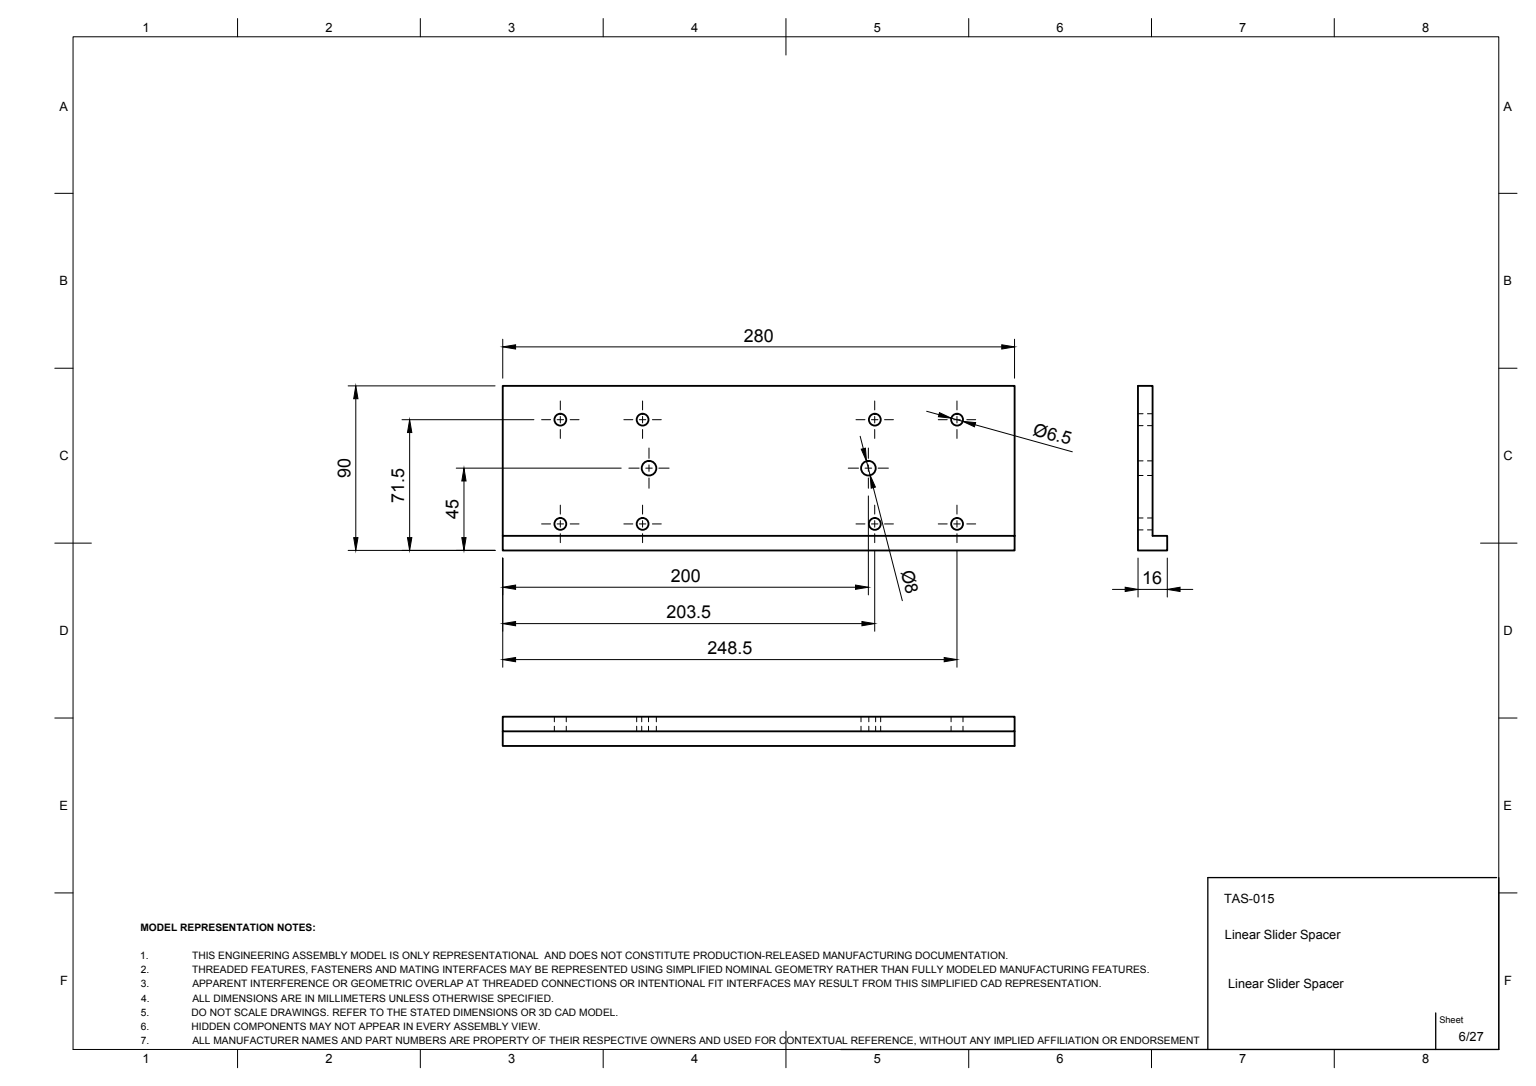
ISO-10303-21;
HEADER;
/* Generated by software containing ST-Developer
 * from STEP Tools, Inc. (www.steptools.com) 
 */

FILE_DESCRIPTION(
/* description */ ('STEP AP214'),
/* implementation_level */ '2;1');

FILE_NAME(
/* name */ 'Linear Slider Spacer.step',
/* time_stamp */ '2026-11-15T14:49:54-08:00',
/* author */ (''),
/* organization */ (''),
/* preprocessor_version */ 'ST-DEVELOPER v20.2',
/* originating_system */ 'Autodesk Translation Framework v15.17.0.0',
/* authorisation */ '');

FILE_SCHEMA (('AUTOMOTIVE_DESIGN { 1 0 10303 214 3 1 1 }'));
ENDSEC;

DATA;
#10=MECHANICAL_DESIGN_GEOMETRIC_PRESENTATION_REPRESENTATION('',(#1131),#66721);
#1065=SHAPE_REPRESENTATION_RELATIONSHIP('SRR','None',#66928,#1096);
#1096=ADVANCED_BREP_SHAPE_REPRESENTATION('',(#1166),#66719);
#1131=STYLED_ITEM('',(#67095),#1166);
#1166=MANIFOLD_SOLID_BREP('Body1',#25697);
#1476=FACE_BOUND('',#5440,.T.);
#1477=FACE_BOUND('',#5441,.T.);
#1478=FACE_BOUND('',#5442,.T.);
#1479=FACE_BOUND('',#5443,.T.);
#1480=FACE_BOUND('',#5444,.T.);
#1481=FACE_BOUND('',#5445,.T.);
#1482=FACE_BOUND('',#5446,.T.);
#1483=FACE_BOUND('',#5447,.T.);
#1484=FACE_BOUND('',#5448,.T.);
#1485=FACE_BOUND('',#5449,.T.);
#1486=FACE_BOUND('',#5455,.T.);
#1487=FACE_BOUND('',#5456,.T.);
#1488=FACE_BOUND('',#5457,.T.);
#1489=FACE_BOUND('',#5458,.T.);
#1490=FACE_BOUND('',#5459,.T.);
#1491=FACE_BOUND('',#5460,.T.);
#1492=FACE_BOUND('',#5461,.T.);
#1493=FACE_BOUND('',#5462,.T.);
#1494=FACE_BOUND('',#5463,.T.);
#1495=FACE_BOUND('',#5464,.T.);
#2251=PLANE('',#28672);
#2252=PLANE('',#28673);
#2253=PLANE('',#28674);
#2254=PLANE('',#28675);
#2255=PLANE('',#28676);
#2256=PLANE('',#28677);
#2257=PLANE('',#28678);
#2258=PLANE('',#28679);
#3679=FACE_OUTER_BOUND('',#5429,.T.);
#3680=FACE_OUTER_BOUND('',#5430,.T.);
#3681=FACE_OUTER_BOUND('',#5431,.T.);
#3682=FACE_OUTER_BOUND('',#5432,.T.);
#3683=FACE_OUTER_BOUND('',#5433,.T.);
#3684=FACE_OUTER_BOUND('',#5434,.T.);
#3685=FACE_OUTER_BOUND('',#5435,.T.);
#3686=FACE_OUTER_BOUND('',#5436,.T.);
#3687=FACE_OUTER_BOUND('',#5437,.T.);
#3688=FACE_OUTER_BOUND('',#5438,.T.);
#3689=FACE_OUTER_BOUND('',#5439,.T.);
#3690=FACE_OUTER_BOUND('',#5450,.T.);
#3691=FACE_OUTER_BOUND('',#5451,.T.);
#3692=FACE_OUTER_BOUND('',#5452,.T.);
#3693=FACE_OUTER_BOUND('',#5453,.T.);
#3694=FACE_OUTER_BOUND('',#5454,.T.);
#3695=FACE_OUTER_BOUND('',#5465,.T.);
#3696=FACE_OUTER_BOUND('',#5466,.T.);
#5429=EDGE_LOOP('',(#23648,#23649,#23650,#23651));
#5430=EDGE_LOOP('',(#23652,#23653,#23654,#23655));
#5431=EDGE_LOOP('',(#23656,#23657,#23658,#23659));
#5432=EDGE_LOOP('',(#23660,#23661,#23662,#23663));
#5433=EDGE_LOOP('',(#23664,#23665,#23666,#23667));
#5434=EDGE_LOOP('',(#23668,#23669,#23670,#23671));
#5435=EDGE_LOOP('',(#23672,#23673,#23674,#23675));
#5436=EDGE_LOOP('',(#23676,#23677,#23678,#23679));
#5437=EDGE_LOOP('',(#23680,#23681,#23682,#23683));
#5438=EDGE_LOOP('',(#23684,#23685,#23686,#23687));
#5439=EDGE_LOOP('',(#23688,#23689,#23690,#23691));
#5440=EDGE_LOOP('',(#23692));
#5441=EDGE_LOOP('',(#23693));
#5442=EDGE_LOOP('',(#23694));
#5443=EDGE_LOOP('',(#23695));
#5444=EDGE_LOOP('',(#23696));
#5445=EDGE_LOOP('',(#23697));
#5446=EDGE_LOOP('',(#23698));
#5447=EDGE_LOOP('',(#23699));
#5448=EDGE_LOOP('',(#23700));
#5449=EDGE_LOOP('',(#23701));
#5450=EDGE_LOOP('',(#23702,#23703,#23704,#23705));
#5451=EDGE_LOOP('',(#23706,#23707,#23708,#23709,#23710,#23711));
#5452=EDGE_LOOP('',(#23712,#23713,#23714,#23715));
#5453=EDGE_LOOP('',(#23716,#23717,#23718,#23719,#23720,#23721));
#5454=EDGE_LOOP('',(#23722,#23723,#23724,#23725));
#5455=EDGE_LOOP('',(#23726));
#5456=EDGE_LOOP('',(#23727));
#5457=EDGE_LOOP('',(#23728));
#5458=EDGE_LOOP('',(#23729));
#5459=EDGE_LOOP('',(#23730));
#5460=EDGE_LOOP('',(#23731));
#5461=EDGE_LOOP('',(#23732));
#5462=EDGE_LOOP('',(#23733));
#5463=EDGE_LOOP('',(#23734));
#5464=EDGE_LOOP('',(#23735));
#5465=EDGE_LOOP('',(#23736,#23737,#23738,#23739));
#5466=EDGE_LOOP('',(#23740,#23741,#23742,#23743));
#7422=LINE('',#66429,#9411);
#7423=LINE('',#66435,#9412);
#7424=LINE('',#66441,#9413);
#7425=LINE('',#66447,#9414);
#7426=LINE('',#66453,#9415);
#7427=LINE('',#66459,#9416);
#7428=LINE('',#66465,#9417);
#7429=LINE('',#66471,#9418);
#7430=LINE('',#66477,#9419);
#7431=LINE('',#66483,#9420);
#7432=LINE('',#66488,#9421);
#7433=LINE('',#66490,#9422);
#7434=LINE('',#66492,#9423);
#7435=LINE('',#66493,#9424);
#7436=LINE('',#66496,#9425);
#7437=LINE('',#66498,#9426);
#7438=LINE('',#66499,#9427);
#7439=LINE('',#66502,#9428);
#7440=LINE('',#66504,#9429);
#7441=LINE('',#66506,#9430);
#7442=LINE('',#66507,#9431);
#7443=LINE('',#66510,#9432);
#7444=LINE('',#66512,#9433);
#7445=LINE('',#66513,#9434);
#7446=LINE('',#66516,#9435);
#7447=LINE('',#66517,#9436);
#7448=LINE('',#66518,#9437);
#7449=LINE('',#66521,#9438);
#9411=VECTOR('',#35901,4.);
#9412=VECTOR('',#35908,4.);
#9413=VECTOR('',#35915,3.25);
#9414=VECTOR('',#35922,3.25);
#9415=VECTOR('',#35929,3.25);
#9416=VECTOR('',#35936,3.25);
#9417=VECTOR('',#35943,3.25);
#9418=VECTOR('',#35950,3.25);
#9419=VECTOR('',#35957,3.25);
#9420=VECTOR('',#35964,3.25);
#9421=VECTOR('',#35969,1000.);
#9422=VECTOR('',#35970,1000.);
#9423=VECTOR('',#35971,1000.);
#9424=VECTOR('',#35972,1000.);
#9425=VECTOR('',#35975,1000.);
#9426=VECTOR('',#35976,1000.);
#9427=VECTOR('',#35977,1000.);
#9428=VECTOR('',#35980,1000.);
#9429=VECTOR('',#35981,1000.);
#9430=VECTOR('',#35982,1000.);
#9431=VECTOR('',#35983,1000.);
#9432=VECTOR('',#35986,1000.);
#9433=VECTOR('',#35987,1000.);
#9434=VECTOR('',#35988,1000.);
#9435=VECTOR('',#35991,1000.);
#9436=VECTOR('',#35992,1000.);
#9437=VECTOR('',#35993,1000.);
#9438=VECTOR('',#35998,1000.);
#10611=CIRCLE('',#28643,4.);
#10612=CIRCLE('',#28644,4.);
#10613=CIRCLE('',#28646,4.);
#10614=CIRCLE('',#28647,4.);
#10615=CIRCLE('',#28649,3.25);
#10616=CIRCLE('',#28650,3.25);
#10617=CIRCLE('',#28652,3.25);
#10618=CIRCLE('',#28653,3.25);
#10619=CIRCLE('',#28655,3.25);
#10620=CIRCLE('',#28656,3.25);
#10621=CIRCLE('',#28658,3.25);
#10622=CIRCLE('',#28659,3.25);
#10623=CIRCLE('',#28661,3.25);
#10624=CIRCLE('',#28662,3.25);
#10625=CIRCLE('',#28664,3.25);
#10626=CIRCLE('',#28665,3.25);
#10627=CIRCLE('',#28667,3.25);
#10628=CIRCLE('',#28668,3.25);
#10629=CIRCLE('',#28670,3.25);
#10630=CIRCLE('',#28671,3.25);
#12939=VERTEX_POINT('',#66426);
#12940=VERTEX_POINT('',#66428);
#12941=VERTEX_POINT('',#66432);
#12942=VERTEX_POINT('',#66434);
#12943=VERTEX_POINT('',#66438);
#12944=VERTEX_POINT('',#66440);
#12945=VERTEX_POINT('',#66444);
#12946=VERTEX_POINT('',#66446);
#12947=VERTEX_POINT('',#66450);
#12948=VERTEX_POINT('',#66452);
#12949=VERTEX_POINT('',#66456);
#12950=VERTEX_POINT('',#66458);
#12951=VERTEX_POINT('',#66462);
#12952=VERTEX_POINT('',#66464);
#12953=VERTEX_POINT('',#66468);
#12954=VERTEX_POINT('',#66470);
#12955=VERTEX_POINT('',#66474);
#12956=VERTEX_POINT('',#66476);
#12957=VERTEX_POINT('',#66480);
#12958=VERTEX_POINT('',#66482);
#12959=VERTEX_POINT('',#66486);
#12960=VERTEX_POINT('',#66487);
#12961=VERTEX_POINT('',#66489);
#12962=VERTEX_POINT('',#66491);
#12963=VERTEX_POINT('',#66495);
#12964=VERTEX_POINT('',#66497);
#12965=VERTEX_POINT('',#66501);
#12966=VERTEX_POINT('',#66503);
#12967=VERTEX_POINT('',#66505);
#12968=VERTEX_POINT('',#66509);
#12969=VERTEX_POINT('',#66511);
#12970=VERTEX_POINT('',#66515);
#16517=EDGE_CURVE('',#12939,#12939,#10611,.T.);
#16518=EDGE_CURVE('',#12939,#12940,#7422,.T.);
#16519=EDGE_CURVE('',#12940,#12940,#10612,.T.);
#16520=EDGE_CURVE('',#12941,#12941,#10613,.T.);
#16521=EDGE_CURVE('',#12941,#12942,#7423,.T.);
#16522=EDGE_CURVE('',#12942,#12942,#10614,.T.);
#16523=EDGE_CURVE('',#12943,#12943,#10615,.T.);
#16524=EDGE_CURVE('',#12943,#12944,#7424,.T.);
#16525=EDGE_CURVE('',#12944,#12944,#10616,.T.);
#16526=EDGE_CURVE('',#12945,#12945,#10617,.T.);
#16527=EDGE_CURVE('',#12945,#12946,#7425,.T.);
#16528=EDGE_CURVE('',#12946,#12946,#10618,.T.);
#16529=EDGE_CURVE('',#12947,#12947,#10619,.T.);
#16530=EDGE_CURVE('',#12947,#12948,#7426,.T.);
#16531=EDGE_CURVE('',#12948,#12948,#10620,.T.);
#16532=EDGE_CURVE('',#12949,#12949,#10621,.T.);
#16533=EDGE_CURVE('',#12949,#12950,#7427,.T.);
#16534=EDGE_CURVE('',#12950,#12950,#10622,.T.);
#16535=EDGE_CURVE('',#12951,#12951,#10623,.T.);
#16536=EDGE_CURVE('',#12951,#12952,#7428,.T.);
#16537=EDGE_CURVE('',#12952,#12952,#10624,.T.);
#16538=EDGE_CURVE('',#12953,#12953,#10625,.T.);
#16539=EDGE_CURVE('',#12953,#12954,#7429,.T.);
#16540=EDGE_CURVE('',#12954,#12954,#10626,.T.);
#16541=EDGE_CURVE('',#12955,#12955,#10627,.T.);
#16542=EDGE_CURVE('',#12955,#12956,#7430,.T.);
#16543=EDGE_CURVE('',#12956,#12956,#10628,.T.);
#16544=EDGE_CURVE('',#12957,#12957,#10629,.T.);
#16545=EDGE_CURVE('',#12957,#12958,#7431,.T.);
#16546=EDGE_CURVE('',#12958,#12958,#10630,.T.);
#16547=EDGE_CURVE('',#12959,#12960,#7432,.T.);
#16548=EDGE_CURVE('',#12961,#12959,#7433,.T.);
#16549=EDGE_CURVE('',#12962,#12961,#7434,.T.);
#16550=EDGE_CURVE('',#12960,#12962,#7435,.T.);
#16551=EDGE_CURVE('',#12963,#12961,#7436,.T.);
#16552=EDGE_CURVE('',#12964,#12963,#7437,.T.);
#16553=EDGE_CURVE('',#12964,#12962,#7438,.T.);
#16554=EDGE_CURVE('',#12959,#12965,#7439,.T.);
#16555=EDGE_CURVE('',#12965,#12966,#7440,.T.);
#16556=EDGE_CURVE('',#12967,#12966,#7441,.T.);
#16557=EDGE_CURVE('',#12963,#12967,#7442,.T.);
#16558=EDGE_CURVE('',#12966,#12968,#7443,.T.);
#16559=EDGE_CURVE('',#12969,#12968,#7444,.T.);
#16560=EDGE_CURVE('',#12967,#12969,#7445,.T.);
#16561=EDGE_CURVE('',#12968,#12970,#7446,.T.);
#16562=EDGE_CURVE('',#12970,#12960,#7447,.T.);
#16563=EDGE_CURVE('',#12969,#12964,#7448,.T.);
#16564=EDGE_CURVE('',#12965,#12970,#7449,.T.);
#23648=ORIENTED_EDGE('',*,*,#16517,.F.);
#23649=ORIENTED_EDGE('',*,*,#16518,.T.);
#23650=ORIENTED_EDGE('',*,*,#16519,.T.);
#23651=ORIENTED_EDGE('',*,*,#16518,.F.);
#23652=ORIENTED_EDGE('',*,*,#16520,.F.);
#23653=ORIENTED_EDGE('',*,*,#16521,.T.);
#23654=ORIENTED_EDGE('',*,*,#16522,.T.);
#23655=ORIENTED_EDGE('',*,*,#16521,.F.);
#23656=ORIENTED_EDGE('',*,*,#16523,.F.);
#23657=ORIENTED_EDGE('',*,*,#16524,.T.);
#23658=ORIENTED_EDGE('',*,*,#16525,.T.);
#23659=ORIENTED_EDGE('',*,*,#16524,.F.);
#23660=ORIENTED_EDGE('',*,*,#16526,.F.);
#23661=ORIENTED_EDGE('',*,*,#16527,.T.);
#23662=ORIENTED_EDGE('',*,*,#16528,.T.);
#23663=ORIENTED_EDGE('',*,*,#16527,.F.);
#23664=ORIENTED_EDGE('',*,*,#16529,.F.);
#23665=ORIENTED_EDGE('',*,*,#16530,.T.);
#23666=ORIENTED_EDGE('',*,*,#16531,.T.);
#23667=ORIENTED_EDGE('',*,*,#16530,.F.);
#23668=ORIENTED_EDGE('',*,*,#16532,.F.);
#23669=ORIENTED_EDGE('',*,*,#16533,.T.);
#23670=ORIENTED_EDGE('',*,*,#16534,.T.);
#23671=ORIENTED_EDGE('',*,*,#16533,.F.);
#23672=ORIENTED_EDGE('',*,*,#16535,.F.);
#23673=ORIENTED_EDGE('',*,*,#16536,.T.);
#23674=ORIENTED_EDGE('',*,*,#16537,.T.);
#23675=ORIENTED_EDGE('',*,*,#16536,.F.);
#23676=ORIENTED_EDGE('',*,*,#16538,.F.);
#23677=ORIENTED_EDGE('',*,*,#16539,.T.);
#23678=ORIENTED_EDGE('',*,*,#16540,.T.);
#23679=ORIENTED_EDGE('',*,*,#16539,.F.);
#23680=ORIENTED_EDGE('',*,*,#16541,.F.);
#23681=ORIENTED_EDGE('',*,*,#16542,.T.);
#23682=ORIENTED_EDGE('',*,*,#16543,.T.);
#23683=ORIENTED_EDGE('',*,*,#16542,.F.);
#23684=ORIENTED_EDGE('',*,*,#16544,.F.);
#23685=ORIENTED_EDGE('',*,*,#16545,.T.);
#23686=ORIENTED_EDGE('',*,*,#16546,.T.);
#23687=ORIENTED_EDGE('',*,*,#16545,.F.);
#23688=ORIENTED_EDGE('',*,*,#16547,.F.);
#23689=ORIENTED_EDGE('',*,*,#16548,.F.);
#23690=ORIENTED_EDGE('',*,*,#16549,.F.);
#23691=ORIENTED_EDGE('',*,*,#16550,.F.);
#23692=ORIENTED_EDGE('',*,*,#16517,.T.);
#23693=ORIENTED_EDGE('',*,*,#16520,.T.);
#23694=ORIENTED_EDGE('',*,*,#16523,.T.);
#23695=ORIENTED_EDGE('',*,*,#16526,.T.);
#23696=ORIENTED_EDGE('',*,*,#16529,.T.);
#23697=ORIENTED_EDGE('',*,*,#16532,.T.);
#23698=ORIENTED_EDGE('',*,*,#16535,.T.);
#23699=ORIENTED_EDGE('',*,*,#16538,.T.);
#23700=ORIENTED_EDGE('',*,*,#16541,.T.);
#23701=ORIENTED_EDGE('',*,*,#16544,.T.);
#23702=ORIENTED_EDGE('',*,*,#16549,.T.);
#23703=ORIENTED_EDGE('',*,*,#16551,.F.);
#23704=ORIENTED_EDGE('',*,*,#16552,.F.);
#23705=ORIENTED_EDGE('',*,*,#16553,.T.);
#23706=ORIENTED_EDGE('',*,*,#16548,.T.);
#23707=ORIENTED_EDGE('',*,*,#16554,.T.);
#23708=ORIENTED_EDGE('',*,*,#16555,.T.);
#23709=ORIENTED_EDGE('',*,*,#16556,.F.);
#23710=ORIENTED_EDGE('',*,*,#16557,.F.);
#23711=ORIENTED_EDGE('',*,*,#16551,.T.);
#23712=ORIENTED_EDGE('',*,*,#16556,.T.);
#23713=ORIENTED_EDGE('',*,*,#16558,.T.);
#23714=ORIENTED_EDGE('',*,*,#16559,.F.);
#23715=ORIENTED_EDGE('',*,*,#16560,.F.);
#23716=ORIENTED_EDGE('',*,*,#16559,.T.);
#23717=ORIENTED_EDGE('',*,*,#16561,.T.);
#23718=ORIENTED_EDGE('',*,*,#16562,.T.);
#23719=ORIENTED_EDGE('',*,*,#16550,.T.);
#23720=ORIENTED_EDGE('',*,*,#16553,.F.);
#23721=ORIENTED_EDGE('',*,*,#16563,.F.);
#23722=ORIENTED_EDGE('',*,*,#16552,.T.);
#23723=ORIENTED_EDGE('',*,*,#16557,.T.);
#23724=ORIENTED_EDGE('',*,*,#16560,.T.);
#23725=ORIENTED_EDGE('',*,*,#16563,.T.);
#23726=ORIENTED_EDGE('',*,*,#16519,.F.);
#23727=ORIENTED_EDGE('',*,*,#16522,.F.);
#23728=ORIENTED_EDGE('',*,*,#16525,.F.);
#23729=ORIENTED_EDGE('',*,*,#16528,.F.);
#23730=ORIENTED_EDGE('',*,*,#16531,.F.);
#23731=ORIENTED_EDGE('',*,*,#16534,.F.);
#23732=ORIENTED_EDGE('',*,*,#16537,.F.);
#23733=ORIENTED_EDGE('',*,*,#16540,.F.);
#23734=ORIENTED_EDGE('',*,*,#16543,.F.);
#23735=ORIENTED_EDGE('',*,*,#16546,.F.);
#23736=ORIENTED_EDGE('',*,*,#16554,.F.);
#23737=ORIENTED_EDGE('',*,*,#16547,.T.);
#23738=ORIENTED_EDGE('',*,*,#16562,.F.);
#23739=ORIENTED_EDGE('',*,*,#16564,.F.);
#23740=ORIENTED_EDGE('',*,*,#16555,.F.);
#23741=ORIENTED_EDGE('',*,*,#16564,.T.);
#23742=ORIENTED_EDGE('',*,*,#16561,.F.);
#23743=ORIENTED_EDGE('',*,*,#16558,.F.);
#24210=CYLINDRICAL_SURFACE('',#28642,4.);
#24211=CYLINDRICAL_SURFACE('',#28645,4.);
#24212=CYLINDRICAL_SURFACE('',#28648,3.25);
#24213=CYLINDRICAL_SURFACE('',#28651,3.25);
#24214=CYLINDRICAL_SURFACE('',#28654,3.25);
#24215=CYLINDRICAL_SURFACE('',#28657,3.25);
#24216=CYLINDRICAL_SURFACE('',#28660,3.25);
#24217=CYLINDRICAL_SURFACE('',#28663,3.25);
#24218=CYLINDRICAL_SURFACE('',#28666,3.25);
#24219=CYLINDRICAL_SURFACE('',#28669,3.25);
#25632=ADVANCED_FACE('',(#3679),#24210,.F.);
#25633=ADVANCED_FACE('',(#3680),#24211,.F.);
#25634=ADVANCED_FACE('',(#3681),#24212,.F.);
#25635=ADVANCED_FACE('',(#3682),#24213,.F.);
#25636=ADVANCED_FACE('',(#3683),#24214,.F.);
#25637=ADVANCED_FACE('',(#3684),#24215,.F.);
#25638=ADVANCED_FACE('',(#3685),#24216,.F.);
#25639=ADVANCED_FACE('',(#3686),#24217,.F.);
#25640=ADVANCED_FACE('',(#3687),#24218,.F.);
#25641=ADVANCED_FACE('',(#3688),#24219,.F.);
#25642=ADVANCED_FACE('',(#3689,#1476,#1477,#1478,#1479,#1480,#1481,#1482,
#1483,#1484,#1485),#2251,.F.);
#25643=ADVANCED_FACE('',(#3690),#2252,.F.);
#25644=ADVANCED_FACE('',(#3691),#2253,.F.);
#25645=ADVANCED_FACE('',(#3692),#2254,.F.);
#25646=ADVANCED_FACE('',(#3693),#2255,.F.);
#25647=ADVANCED_FACE('',(#3694,#1486,#1487,#1488,#1489,#1490,#1491,#1492,
#1493,#1494,#1495),#2256,.T.);
#25648=ADVANCED_FACE('',(#3695),#2257,.T.);
#25649=ADVANCED_FACE('',(#3696),#2258,.T.);
#25697=CLOSED_SHELL('',(#25632,#25633,#25634,#25635,#25636,#25637,#25638,
#25639,#25640,#25641,#25642,#25643,#25644,#25645,#25646,#25647,#25648,#25649));
#28641=AXIS2_PLACEMENT_3D('',#66424,#35895,#35896);
#28642=AXIS2_PLACEMENT_3D('',#66425,#35897,#35898);
#28643=AXIS2_PLACEMENT_3D('',#66427,#35899,#35900);
#28644=AXIS2_PLACEMENT_3D('',#66430,#35902,#35903);
#28645=AXIS2_PLACEMENT_3D('',#66431,#35904,#35905);
#28646=AXIS2_PLACEMENT_3D('',#66433,#35906,#35907);
#28647=AXIS2_PLACEMENT_3D('',#66436,#35909,#35910);
#28648=AXIS2_PLACEMENT_3D('',#66437,#35911,#35912);
#28649=AXIS2_PLACEMENT_3D('',#66439,#35913,#35914);
#28650=AXIS2_PLACEMENT_3D('',#66442,#35916,#35917);
#28651=AXIS2_PLACEMENT_3D('',#66443,#35918,#35919);
#28652=AXIS2_PLACEMENT_3D('',#66445,#35920,#35921);
#28653=AXIS2_PLACEMENT_3D('',#66448,#35923,#35924);
#28654=AXIS2_PLACEMENT_3D('',#66449,#35925,#35926);
#28655=AXIS2_PLACEMENT_3D('',#66451,#35927,#35928);
#28656=AXIS2_PLACEMENT_3D('',#66454,#35930,#35931);
#28657=AXIS2_PLACEMENT_3D('',#66455,#35932,#35933);
#28658=AXIS2_PLACEMENT_3D('',#66457,#35934,#35935);
#28659=AXIS2_PLACEMENT_3D('',#66460,#35937,#35938);
#28660=AXIS2_PLACEMENT_3D('',#66461,#35939,#35940);
#28661=AXIS2_PLACEMENT_3D('',#66463,#35941,#35942);
#28662=AXIS2_PLACEMENT_3D('',#66466,#35944,#35945);
#28663=AXIS2_PLACEMENT_3D('',#66467,#35946,#35947);
#28664=AXIS2_PLACEMENT_3D('',#66469,#35948,#35949);
#28665=AXIS2_PLACEMENT_3D('',#66472,#35951,#35952);
#28666=AXIS2_PLACEMENT_3D('',#66473,#35953,#35954);
#28667=AXIS2_PLACEMENT_3D('',#66475,#35955,#35956);
#28668=AXIS2_PLACEMENT_3D('',#66478,#35958,#35959);
#28669=AXIS2_PLACEMENT_3D('',#66479,#35960,#35961);
#28670=AXIS2_PLACEMENT_3D('',#66481,#35962,#35963);
#28671=AXIS2_PLACEMENT_3D('',#66484,#35965,#35966);
#28672=AXIS2_PLACEMENT_3D('',#66485,#35967,#35968);
#28673=AXIS2_PLACEMENT_3D('',#66494,#35973,#35974);
#28674=AXIS2_PLACEMENT_3D('',#66500,#35978,#35979);
#28675=AXIS2_PLACEMENT_3D('',#66508,#35984,#35985);
#28676=AXIS2_PLACEMENT_3D('',#66514,#35989,#35990);
#28677=AXIS2_PLACEMENT_3D('',#66519,#35994,#35995);
#28678=AXIS2_PLACEMENT_3D('',#66520,#35996,#35997);
#28679=AXIS2_PLACEMENT_3D('',#66522,#35999,#36000);
#35895=DIRECTION('axis',(0.,0.,1.));
#35896=DIRECTION('refdir',(1.,0.,0.));
#35897=DIRECTION('center_axis',(0.,0.,1.));
#35898=DIRECTION('ref_axis',(1.,0.,0.));
#35899=DIRECTION('center_axis',(0.,0.,1.));
#35900=DIRECTION('ref_axis',(1.,0.,0.));
#35901=DIRECTION('',(0.,0.,1.));
#35902=DIRECTION('center_axis',(0.,0.,1.));
#35903=DIRECTION('ref_axis',(1.,0.,0.));
#35904=DIRECTION('center_axis',(0.,0.,1.));
#35905=DIRECTION('ref_axis',(1.,0.,0.));
#35906=DIRECTION('center_axis',(0.,0.,1.));
#35907=DIRECTION('ref_axis',(1.,0.,0.));
#35908=DIRECTION('',(0.,0.,1.));
#35909=DIRECTION('center_axis',(0.,0.,1.));
#35910=DIRECTION('ref_axis',(1.,0.,0.));
#35911=DIRECTION('center_axis',(0.,0.,1.));
#35912=DIRECTION('ref_axis',(1.,0.,0.));
#35913=DIRECTION('center_axis',(0.,0.,1.));
#35914=DIRECTION('ref_axis',(1.,0.,0.));
#35915=DIRECTION('',(0.,0.,1.));
#35916=DIRECTION('center_axis',(0.,0.,1.));
#35917=DIRECTION('ref_axis',(1.,0.,0.));
#35918=DIRECTION('center_axis',(0.,0.,1.));
#35919=DIRECTION('ref_axis',(1.,0.,0.));
#35920=DIRECTION('center_axis',(0.,0.,1.));
#35921=DIRECTION('ref_axis',(1.,0.,0.));
#35922=DIRECTION('',(0.,0.,1.));
#35923=DIRECTION('center_axis',(0.,0.,1.));
#35924=DIRECTION('ref_axis',(1.,0.,0.));
#35925=DIRECTION('center_axis',(0.,0.,1.));
#35926=DIRECTION('ref_axis',(1.,0.,0.));
#35927=DIRECTION('center_axis',(0.,0.,1.));
#35928=DIRECTION('ref_axis',(1.,0.,0.));
#35929=DIRECTION('',(0.,0.,1.));
#35930=DIRECTION('center_axis',(0.,0.,1.));
#35931=DIRECTION('ref_axis',(1.,0.,0.));
#35932=DIRECTION('center_axis',(0.,0.,1.));
#35933=DIRECTION('ref_axis',(1.,0.,0.));
#35934=DIRECTION('center_axis',(0.,0.,1.));
#35935=DIRECTION('ref_axis',(1.,0.,0.));
#35936=DIRECTION('',(0.,0.,1.));
#35937=DIRECTION('center_axis',(0.,0.,1.));
#35938=DIRECTION('ref_axis',(1.,0.,0.));
#35939=DIRECTION('center_axis',(0.,0.,1.));
#35940=DIRECTION('ref_axis',(1.,0.,0.));
#35941=DIRECTION('center_axis',(0.,0.,1.));
#35942=DIRECTION('ref_axis',(1.,0.,0.));
#35943=DIRECTION('',(0.,0.,1.));
#35944=DIRECTION('center_axis',(0.,0.,1.));
#35945=DIRECTION('ref_axis',(1.,0.,0.));
#35946=DIRECTION('center_axis',(0.,0.,1.));
#35947=DIRECTION('ref_axis',(1.,0.,0.));
#35948=DIRECTION('center_axis',(0.,0.,1.));
#35949=DIRECTION('ref_axis',(1.,0.,0.));
#35950=DIRECTION('',(0.,0.,1.));
#35951=DIRECTION('center_axis',(0.,0.,1.));
#35952=DIRECTION('ref_axis',(1.,0.,0.));
#35953=DIRECTION('center_axis',(0.,0.,1.));
#35954=DIRECTION('ref_axis',(1.,0.,0.));
#35955=DIRECTION('center_axis',(0.,0.,1.));
#35956=DIRECTION('ref_axis',(1.,0.,0.));
#35957=DIRECTION('',(0.,0.,1.));
#35958=DIRECTION('center_axis',(0.,0.,1.));
#35959=DIRECTION('ref_axis',(1.,0.,0.));
#35960=DIRECTION('center_axis',(0.,0.,1.));
#35961=DIRECTION('ref_axis',(1.,0.,0.));
#35962=DIRECTION('center_axis',(0.,0.,1.));
#35963=DIRECTION('ref_axis',(1.,0.,0.));
#35964=DIRECTION('',(0.,0.,1.));
#35965=DIRECTION('center_axis',(0.,0.,1.));
#35966=DIRECTION('ref_axis',(1.,0.,0.));
#35967=DIRECTION('center_axis',(0.,0.,1.));
#35968=DIRECTION('ref_axis',(1.,0.,0.));
#35969=DIRECTION('',(0.,-1.,0.));
#35970=DIRECTION('',(-1.,0.,0.));
#35971=DIRECTION('',(-1.23908819712629E-16,1.,0.));
#35972=DIRECTION('',(1.,0.,0.));
#35973=DIRECTION('center_axis',(-1.,-1.23908819712629E-16,0.));
#35974=DIRECTION('ref_axis',(1.23908819712629E-16,-1.,0.));
#35975=DIRECTION('',(0.,0.,-1.));
#35976=DIRECTION('',(-1.23908819712629E-16,1.,0.));
#35977=DIRECTION('',(0.,0.,-1.));
#35978=DIRECTION('center_axis',(0.,-1.,0.));
#35979=DIRECTION('ref_axis',(0.,0.,-1.));
#35980=DIRECTION('',(0.,0.,-1.));
#35981=DIRECTION('',(-1.,0.,0.));
#35982=DIRECTION('',(0.,0.,-1.));
#35983=DIRECTION('',(-1.,0.,0.));
#35984=DIRECTION('center_axis',(1.,1.23908819712629E-16,0.));
#35985=DIRECTION('ref_axis',(-1.23908819712629E-16,1.,0.));
#35986=DIRECTION('',(0.,-1.,0.));
#35987=DIRECTION('',(0.,0.,-1.));
#35988=DIRECTION('',(1.23908819712629E-16,-1.,0.));
#35989=DIRECTION('center_axis',(0.,1.,0.));
#35990=DIRECTION('ref_axis',(0.,0.,1.));
#35991=DIRECTION('',(1.,0.,0.));
#35992=DIRECTION('',(0.,0.,1.));
#35993=DIRECTION('',(1.,0.,0.));
#35994=DIRECTION('center_axis',(0.,0.,1.));
#35995=DIRECTION('ref_axis',(1.,0.,0.));
#35996=DIRECTION('center_axis',(1.,0.,0.));
#35997=DIRECTION('ref_axis',(0.,0.,-1.));
#35998=DIRECTION('',(0.,-1.,0.));
#35999=DIRECTION('center_axis',(0.,0.,-1.));
#36000=DIRECTION('ref_axis',(-1.,0.,0.));
#66424=CARTESIAN_POINT('',(0.,0.,0.));
#66425=CARTESIAN_POINT('Origin',(0.,-60.,8.));
#66426=CARTESIAN_POINT('',(-4.,-60.,0.));
#66427=CARTESIAN_POINT('Origin',(0.,-60.,0.));
#66428=CARTESIAN_POINT('',(-4.,-60.,8.));
#66429=CARTESIAN_POINT('',(-4.,-60.,8.));
#66430=CARTESIAN_POINT('Origin',(0.,-60.,8.));
#66431=CARTESIAN_POINT('Origin',(0.,60.,8.));
#66432=CARTESIAN_POINT('',(-4.,60.,0.));
#66433=CARTESIAN_POINT('Origin',(0.,60.,0.));
#66434=CARTESIAN_POINT('',(-4.,60.,8.));
#66435=CARTESIAN_POINT('',(-4.,60.,8.));
#66436=CARTESIAN_POINT('Origin',(0.,60.,8.));
#66437=CARTESIAN_POINT('Origin',(-30.5,-108.5,8.));
#66438=CARTESIAN_POINT('',(-33.75,-108.5,0.));
#66439=CARTESIAN_POINT('Origin',(-30.5,-108.5,0.));
#66440=CARTESIAN_POINT('',(-33.75,-108.5,8.));
#66441=CARTESIAN_POINT('',(-33.75,-108.5,8.));
#66442=CARTESIAN_POINT('Origin',(-30.5,-108.5,8.));
#66443=CARTESIAN_POINT('Origin',(-30.5,-63.5,8.));
#66444=CARTESIAN_POINT('',(-33.75,-63.5,0.));
#66445=CARTESIAN_POINT('Origin',(-30.5,-63.5,0.));
#66446=CARTESIAN_POINT('',(-33.75,-63.5,8.));
#66447=CARTESIAN_POINT('',(-33.75,-63.5,8.));
#66448=CARTESIAN_POINT('Origin',(-30.5,-63.5,8.));
#66449=CARTESIAN_POINT('Origin',(26.5,-108.5,8.));
#66450=CARTESIAN_POINT('',(23.25,-108.5,0.));
#66451=CARTESIAN_POINT('Origin',(26.5,-108.5,0.));
#66452=CARTESIAN_POINT('',(23.25,-108.5,8.));
#66453=CARTESIAN_POINT('',(23.25,-108.5,8.));
#66454=CARTESIAN_POINT('Origin',(26.5,-108.5,8.));
#66455=CARTESIAN_POINT('Origin',(26.5,-63.5,8.));
#66456=CARTESIAN_POINT('',(23.25,-63.5,0.));
#66457=CARTESIAN_POINT('Origin',(26.5,-63.5,0.));
#66458=CARTESIAN_POINT('',(23.25,-63.5,8.));
#66459=CARTESIAN_POINT('',(23.25,-63.5,8.));
#66460=CARTESIAN_POINT('Origin',(26.5,-63.5,8.));
#66461=CARTESIAN_POINT('Origin',(-30.5,63.5,8.));
#66462=CARTESIAN_POINT('',(-33.75,63.5,0.));
#66463=CARTESIAN_POINT('Origin',(-30.5,63.5,0.));
#66464=CARTESIAN_POINT('',(-33.75,63.5,8.));
#66465=CARTESIAN_POINT('',(-33.75,63.5,8.));
#66466=CARTESIAN_POINT('Origin',(-30.5,63.5,8.));
#66467=CARTESIAN_POINT('Origin',(-30.5,108.5,8.));
#66468=CARTESIAN_POINT('',(-33.75,108.5,0.));
#66469=CARTESIAN_POINT('Origin',(-30.5,108.5,0.));
#66470=CARTESIAN_POINT('',(-33.75,108.5,8.));
#66471=CARTESIAN_POINT('',(-33.75,108.5,8.));
#66472=CARTESIAN_POINT('Origin',(-30.5,108.5,8.));
#66473=CARTESIAN_POINT('Origin',(26.5,63.5,8.));
#66474=CARTESIAN_POINT('',(23.25,63.5,0.));
#66475=CARTESIAN_POINT('Origin',(26.5,63.5,0.));
#66476=CARTESIAN_POINT('',(23.25,63.5,8.));
#66477=CARTESIAN_POINT('',(23.25,63.5,8.));
#66478=CARTESIAN_POINT('Origin',(26.5,63.5,8.));
#66479=CARTESIAN_POINT('Origin',(26.5,108.5,8.));
#66480=CARTESIAN_POINT('',(23.25,108.5,0.));
#66481=CARTESIAN_POINT('Origin',(26.5,108.5,0.));
#66482=CARTESIAN_POINT('',(23.25,108.5,8.));
#66483=CARTESIAN_POINT('',(23.25,108.5,8.));
#66484=CARTESIAN_POINT('Origin',(26.5,108.5,8.));
#66485=CARTESIAN_POINT('Origin',(0.,0.,0.));
#66486=CARTESIAN_POINT('',(-37.,140.,0.));
#66487=CARTESIAN_POINT('',(-37.,-140.,0.));
#66488=CARTESIAN_POINT('',(-37.,151.313708498985,0.));
#66489=CARTESIAN_POINT('',(45.,140.,0.));
#66490=CARTESIAN_POINT('',(-45.,140.,0.));
#66491=CARTESIAN_POINT('',(45.,-140.,0.));
#66492=CARTESIAN_POINT('',(45.,140.,0.));
#66493=CARTESIAN_POINT('',(-45.,-140.,0.));
#66494=CARTESIAN_POINT('Origin',(45.,140.,8.));
#66495=CARTESIAN_POINT('',(45.,140.,8.));
#66496=CARTESIAN_POINT('',(45.,140.,8.));
#66497=CARTESIAN_POINT('',(45.,-140.,8.));
#66498=CARTESIAN_POINT('',(45.,140.,8.));
#66499=CARTESIAN_POINT('',(45.,-140.,8.));
#66500=CARTESIAN_POINT('Origin',(-45.,140.,8.));
#66501=CARTESIAN_POINT('',(-37.,140.,-8.));
#66502=CARTESIAN_POINT('',(-37.,140.,0.));
#66503=CARTESIAN_POINT('',(-45.,140.,-8.));
#66504=CARTESIAN_POINT('',(-45.,140.,-8.));
#66505=CARTESIAN_POINT('',(-45.,140.,8.));
#66506=CARTESIAN_POINT('',(-45.,140.,8.));
#66507=CARTESIAN_POINT('',(-45.,140.,8.));
#66508=CARTESIAN_POINT('Origin',(-45.,140.,8.));
#66509=CARTESIAN_POINT('',(-45.,-140.,-8.));
#66510=CARTESIAN_POINT('',(-45.,151.313708498985,-8.));
#66511=CARTESIAN_POINT('',(-45.,-140.,8.));
#66512=CARTESIAN_POINT('',(-45.,-140.,8.));
#66513=CARTESIAN_POINT('',(-45.,140.,8.));
#66514=CARTESIAN_POINT('Origin',(-45.,-140.,8.));
#66515=CARTESIAN_POINT('',(-37.,-140.,-8.));
#66516=CARTESIAN_POINT('',(-45.,-140.,-8.));
#66517=CARTESIAN_POINT('',(-37.,-140.,0.));
#66518=CARTESIAN_POINT('',(-45.,-140.,8.));
#66519=CARTESIAN_POINT('Origin',(0.,0.,8.));
#66520=CARTESIAN_POINT('Origin',(-37.,151.313708498985,0.));
#66521=CARTESIAN_POINT('',(-37.,151.313708498985,-8.));
#66522=CARTESIAN_POINT('Origin',(-45.,151.313708498985,-8.));
#66678=UNCERTAINTY_MEASURE_WITH_UNIT(LENGTH_MEASURE(0.01),#66722,
'DISTANCE_ACCURACY_VALUE',
'Maximum model space distance between geometric entities at asserted c
onnectivities');
#66680=UNCERTAINTY_MEASURE_WITH_UNIT(LENGTH_MEASURE(0.01),#66722,
'DISTANCE_ACCURACY_VALUE',
'Maximum model space distance between geometric entities at asserted c
onnectivities');
#66719=(
GEOMETRIC_REPRESENTATION_CONTEXT(3)
GLOBAL_UNCERTAINTY_ASSIGNED_CONTEXT((#66678))
GLOBAL_UNIT_ASSIGNED_CONTEXT((#66722,#66724,#66725))
REPRESENTATION_CONTEXT('','3D')
);
#66721=(
GEOMETRIC_REPRESENTATION_CONTEXT(3)
GLOBAL_UNCERTAINTY_ASSIGNED_CONTEXT((#66680))
GLOBAL_UNIT_ASSIGNED_CONTEXT((#66722,#66724,#66725))
REPRESENTATION_CONTEXT('','3D')
);
#66722=(
LENGTH_UNIT()
NAMED_UNIT(*)
SI_UNIT(.MILLI.,.METRE.)
);
#66724=(
NAMED_UNIT(*)
PLANE_ANGLE_UNIT()
SI_UNIT($,.RADIAN.)
);
#66725=(
NAMED_UNIT(*)
SI_UNIT($,.STERADIAN.)
SOLID_ANGLE_UNIT()
);
#66764=SHAPE_DEFINITION_REPRESENTATION(#66834,#66928);
#66834=PRODUCT_DEFINITION_SHAPE('',$,#66969);
#66928=SHAPE_REPRESENTATION('',(#28641),#66719);
#66930=PRODUCT_DEFINITION_CONTEXT('part definition',#67052,'design');
#66969=PRODUCT_DEFINITION('Linear Slider Spacer','Linear Slider Spacer',
#67009,#66930);
#67009=PRODUCT_DEFINITION_FORMATION('',$,#67092);
#67052=APPLICATION_CONTEXT(
'Core Data for Automotive Mechanical Design Process');
#67053=PRODUCT_CONTEXT('part definition',#67052,'mechanical');
#67092=PRODUCT('Linear Slider Spacer','Linear Slider Spacer',$,(#67053));
#67095=PRESENTATION_STYLE_ASSIGNMENT((#67097));
#67097=SURFACE_STYLE_USAGE(.BOTH.,#67099);
#67099=SURFACE_SIDE_STYLE('',(#67101));
#67101=SURFACE_STYLE_FILL_AREA(#67103);
#67103=FILL_AREA_STYLE('Opaque(202,209,238)',(#67105));
#67105=FILL_AREA_STYLE_COLOUR('Opaque(202,209,238)',#67107);
#67107=COLOUR_RGB('Opaque(202,209,238)',0.792156862745098,0.819607843137255,
0.933333333333333);
ENDSEC;
END-ISO-10303-21;
